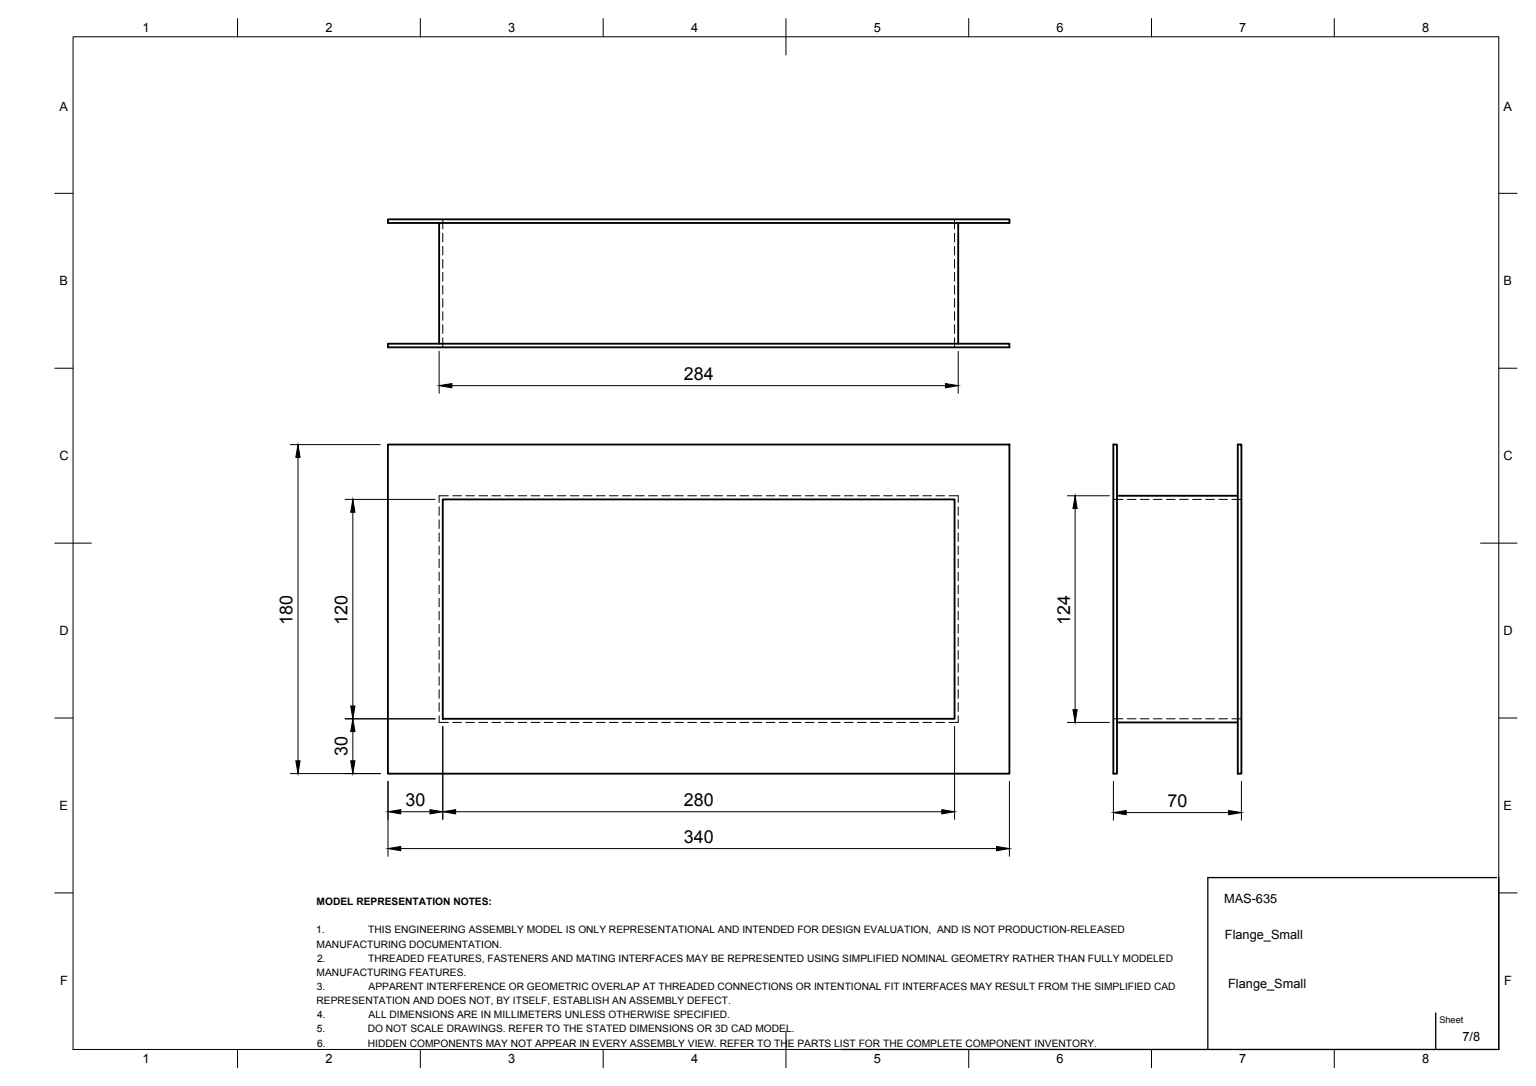
ISO-10303-21;
HEADER;
FILE_DESCRIPTION((''),'2;1');
FILE_NAME('Flange_Small.step','2026-10-09T12:34:24-07:00',(''),(''),'','','');
FILE_SCHEMA (('AUTOMOTIVE_DESIGN { 1 0 10303 214 3 1 1 }'));
ENDSEC;
DATA;
#10=MECHANICAL_DESIGN_GEOMETRIC_PRESENTATION_REPRESENTATION('',(#64),#3759);
#52=SHAPE_REPRESENTATION_RELATIONSHIP('SRR','None',#3793,#58) ;
#58=ADVANCED_BREP_SHAPE_REPRESENTATION('',(#70),#3758) ;
#64=STYLED_ITEM('',(#3827),#70) ;
#70=MANIFOLD_SOLID_BREP('Body1',#2268) ;
#137=FACE_BOUND('',#384,.T.) ;
#138=FACE_BOUND('',#386,.T.) ;
#139=FACE_BOUND('',#396,.T.) ;
#140=FACE_BOUND('',#398,.T.) ;
#241=FACE_OUTER_BOUND('',#379,.T.) ;
#242=FACE_OUTER_BOUND('',#380,.T.) ;
#243=FACE_OUTER_BOUND('',#381,.T.) ;
#244=FACE_OUTER_BOUND('',#382,.T.) ;
#245=FACE_OUTER_BOUND('',#383,.T.) ;
#246=FACE_OUTER_BOUND('',#385,.T.) ;
#247=FACE_OUTER_BOUND('',#387,.T.) ;
#248=FACE_OUTER_BOUND('',#388,.T.) ;
#249=FACE_OUTER_BOUND('',#389,.T.) ;
#250=FACE_OUTER_BOUND('',#390,.T.) ;
#251=FACE_OUTER_BOUND('',#391,.T.) ;
#252=FACE_OUTER_BOUND('',#392,.T.) ;
#253=FACE_OUTER_BOUND('',#393,.T.) ;
#254=FACE_OUTER_BOUND('',#394,.T.) ;
#255=FACE_OUTER_BOUND('',#395,.T.) ;
#256=FACE_OUTER_BOUND('',#397,.T.) ;
#257=FACE_OUTER_BOUND('',#399,.T.) ;
#258=FACE_OUTER_BOUND('',#400,.T.) ;
#259=FACE_OUTER_BOUND('',#401,.T.) ;
#260=FACE_OUTER_BOUND('',#402,.T.) ;
#379=EDGE_LOOP('',(#1943,#1944,#1945,#1946)) ;
#380=EDGE_LOOP('',(#1947,#1948,#1949,#1950)) ;
#381=EDGE_LOOP('',(#1951,#1952,#1953,#1954)) ;
#382=EDGE_LOOP('',(#1955,#1956,#1957,#1958)) ;
#383=EDGE_LOOP('',(#1959,#1960,#1961,#1962)) ;
#384=EDGE_LOOP('',(#1963,#1964,#1965,#1966)) ;
#385=EDGE_LOOP('',(#1967,#1968,#1969,#1970)) ;
#386=EDGE_LOOP('',(#1971,#1972,#1973,#1974)) ;
#387=EDGE_LOOP('',(#1975,#1976,#1977,#1978)) ;
#388=EDGE_LOOP('',(#1979,#1980,#1981,#1982)) ;
#389=EDGE_LOOP('',(#1983,#1984,#1985,#1986)) ;
#390=EDGE_LOOP('',(#1987,#1988,#1989,#1990)) ;
#391=EDGE_LOOP('',(#1991,#1992,#1993,#1994)) ;
#392=EDGE_LOOP('',(#1995,#1996,#1997,#1998)) ;
#393=EDGE_LOOP('',(#1999,#2000,#2001,#2002)) ;
#394=EDGE_LOOP('',(#2003,#2004,#2005,#2006)) ;
#395=EDGE_LOOP('',(#2007,#2008,#2009,#2010)) ;
#396=EDGE_LOOP('',(#2011,#2012,#2013,#2014)) ;
#397=EDGE_LOOP('',(#2015,#2016,#2017,#2018)) ;
#398=EDGE_LOOP('',(#2019,#2020,#2021,#2022)) ;
#399=EDGE_LOOP('',(#2023,#2024,#2025,#2026)) ;
#400=EDGE_LOOP('',(#2027,#2028,#2029,#2030)) ;
#401=EDGE_LOOP('',(#2031,#2032,#2033,#2034)) ;
#402=EDGE_LOOP('',(#2035,#2036,#2037,#2038)) ;
#623=LINE('',#3638,#891) ;
#624=LINE('',#3640,#892) ;
#625=LINE('',#3642,#893) ;
#626=LINE('',#3643,#894) ;
#627=LINE('',#3646,#895) ;
#628=LINE('',#3648,#896) ;
#629=LINE('',#3649,#897) ;
#630=LINE('',#3652,#898) ;
#631=LINE('',#3654,#899) ;
#632=LINE('',#3655,#900) ;
#633=LINE('',#3657,#901) ;
#634=LINE('',#3658,#902) ;
#635=LINE('',#3662,#903) ;
#636=LINE('',#3664,#904) ;
#637=LINE('',#3666,#905) ;
#638=LINE('',#3667,#906) ;
#639=LINE('',#3671,#907) ;
#640=LINE('',#3673,#908) ;
#641=LINE('',#3675,#909) ;
#642=LINE('',#3676,#910) ;
#643=LINE('',#3679,#911) ;
#644=LINE('',#3681,#912) ;
#645=LINE('',#3683,#913) ;
#646=LINE('',#3684,#914) ;
#647=LINE('',#3686,#915) ;
#648=LINE('',#3687,#916) ;
#649=LINE('',#3689,#917) ;
#650=LINE('',#3691,#918) ;
#651=LINE('',#3695,#919) ;
#652=LINE('',#3697,#920) ;
#653=LINE('',#3698,#921) ;
#654=LINE('',#3701,#922) ;
#655=LINE('',#3702,#923) ;
#656=LINE('',#3705,#924) ;
#657=LINE('',#3706,#925) ;
#658=LINE('',#3708,#926) ;
#659=LINE('',#3712,#927) ;
#660=LINE('',#3714,#928) ;
#661=LINE('',#3716,#929) ;
#662=LINE('',#3717,#930) ;
#663=LINE('',#3721,#931) ;
#664=LINE('',#3723,#932) ;
#665=LINE('',#3725,#933) ;
#666=LINE('',#3726,#934) ;
#667=LINE('',#3728,#935) ;
#668=LINE('',#3729,#936) ;
#669=LINE('',#3731,#937) ;
#670=LINE('',#3733,#938) ;
#891=VECTOR('',#3004,100.) ;
#892=VECTOR('',#3005,100.) ;
#893=VECTOR('',#3006,100.) ;
#894=VECTOR('',#3007,100.) ;
#895=VECTOR('',#3010,100.) ;
#896=VECTOR('',#3011,100.) ;
#897=VECTOR('',#3012,100.) ;
#898=VECTOR('',#3015,100.) ;
#899=VECTOR('',#3016,100.) ;
#900=VECTOR('',#3017,100.) ;
#901=VECTOR('',#3020,100.) ;
#902=VECTOR('',#3021,100.) ;
#903=VECTOR('',#3024,100.) ;
#904=VECTOR('',#3025,100.) ;
#905=VECTOR('',#3026,100.) ;
#906=VECTOR('',#3027,100.) ;
#907=VECTOR('',#3030,100.) ;
#908=VECTOR('',#3031,100.) ;
#909=VECTOR('',#3032,100.) ;
#910=VECTOR('',#3033,100.) ;
#911=VECTOR('',#3034,100.) ;
#912=VECTOR('',#3035,100.) ;
#913=VECTOR('',#3036,100.) ;
#914=VECTOR('',#3037,100.) ;
#915=VECTOR('',#3040,100.) ;
#916=VECTOR('',#3041,100.) ;
#917=VECTOR('',#3044,100.) ;
#918=VECTOR('',#3047,100.) ;
#919=VECTOR('',#3052,100.) ;
#920=VECTOR('',#3053,100.) ;
#921=VECTOR('',#3054,100.) ;
#922=VECTOR('',#3057,100.) ;
#923=VECTOR('',#3058,100.) ;
#924=VECTOR('',#3061,100.) ;
#925=VECTOR('',#3062,100.) ;
#926=VECTOR('',#3065,100.) ;
#927=VECTOR('',#3068,100.) ;
#928=VECTOR('',#3069,100.) ;
#929=VECTOR('',#3070,100.) ;
#930=VECTOR('',#3071,100.) ;
#931=VECTOR('',#3074,100.) ;
#932=VECTOR('',#3075,100.) ;
#933=VECTOR('',#3076,100.) ;
#934=VECTOR('',#3077,100.) ;
#935=VECTOR('',#3080,100.) ;
#936=VECTOR('',#3081,100.) ;
#937=VECTOR('',#3084,100.) ;
#938=VECTOR('',#3087,100.) ;
#1107=VERTEX_POINT('',#3636) ;
#1108=VERTEX_POINT('',#3637) ;
#1109=VERTEX_POINT('',#3639) ;
#1110=VERTEX_POINT('',#3641) ;
#1111=VERTEX_POINT('',#3645) ;
#1112=VERTEX_POINT('',#3647) ;
#1113=VERTEX_POINT('',#3651) ;
#1114=VERTEX_POINT('',#3653) ;
#1115=VERTEX_POINT('',#3660) ;
#1116=VERTEX_POINT('',#3661) ;
#1117=VERTEX_POINT('',#3663) ;
#1118=VERTEX_POINT('',#3665) ;
#1119=VERTEX_POINT('',#3669) ;
#1120=VERTEX_POINT('',#3670) ;
#1121=VERTEX_POINT('',#3672) ;
#1122=VERTEX_POINT('',#3674) ;
#1123=VERTEX_POINT('',#3677) ;
#1124=VERTEX_POINT('',#3678) ;
#1125=VERTEX_POINT('',#3680) ;
#1126=VERTEX_POINT('',#3682) ;
#1127=VERTEX_POINT('',#3694) ;
#1128=VERTEX_POINT('',#3696) ;
#1129=VERTEX_POINT('',#3700) ;
#1130=VERTEX_POINT('',#3704) ;
#1131=VERTEX_POINT('',#3710) ;
#1132=VERTEX_POINT('',#3711) ;
#1133=VERTEX_POINT('',#3713) ;
#1134=VERTEX_POINT('',#3715) ;
#1135=VERTEX_POINT('',#3719) ;
#1136=VERTEX_POINT('',#3720) ;
#1137=VERTEX_POINT('',#3722) ;
#1138=VERTEX_POINT('',#3724) ;
#1391=EDGE_CURVE('',#1107,#1108,#623,.T.) ;
#1392=EDGE_CURVE('',#1107,#1109,#624,.T.) ;
#1393=EDGE_CURVE('',#1110,#1109,#625,.T.) ;
#1394=EDGE_CURVE('',#1108,#1110,#626,.T.) ;
#1395=EDGE_CURVE('',#1108,#1111,#627,.T.) ;
#1396=EDGE_CURVE('',#1112,#1110,#628,.T.) ;
#1397=EDGE_CURVE('',#1111,#1112,#629,.T.) ;
#1398=EDGE_CURVE('',#1111,#1113,#630,.T.) ;
#1399=EDGE_CURVE('',#1114,#1112,#631,.T.) ;
#1400=EDGE_CURVE('',#1113,#1114,#632,.T.) ;
#1401=EDGE_CURVE('',#1113,#1107,#633,.T.) ;
#1402=EDGE_CURVE('',#1109,#1114,#634,.T.) ;
#1403=EDGE_CURVE('',#1115,#1116,#635,.T.) ;
#1404=EDGE_CURVE('',#1116,#1117,#636,.T.) ;
#1405=EDGE_CURVE('',#1117,#1118,#637,.T.) ;
#1406=EDGE_CURVE('',#1118,#1115,#638,.T.) ;
#1407=EDGE_CURVE('',#1119,#1120,#639,.T.) ;
#1408=EDGE_CURVE('',#1121,#1119,#640,.T.) ;
#1409=EDGE_CURVE('',#1122,#1121,#641,.T.) ;
#1410=EDGE_CURVE('',#1120,#1122,#642,.T.) ;
#1411=EDGE_CURVE('',#1123,#1124,#643,.T.) ;
#1412=EDGE_CURVE('',#1124,#1125,#644,.T.) ;
#1413=EDGE_CURVE('',#1125,#1126,#645,.T.) ;
#1414=EDGE_CURVE('',#1126,#1123,#646,.T.) ;
#1415=EDGE_CURVE('',#1116,#1120,#647,.T.) ;
#1416=EDGE_CURVE('',#1115,#1119,#648,.T.) ;
#1417=EDGE_CURVE('',#1117,#1122,#649,.T.) ;
#1418=EDGE_CURVE('',#1118,#1121,#650,.T.) ;
#1419=EDGE_CURVE('',#1127,#1124,#651,.T.) ;
#1420=EDGE_CURVE('',#1128,#1123,#652,.T.) ;
#1421=EDGE_CURVE('',#1128,#1127,#653,.T.) ;
#1422=EDGE_CURVE('',#1129,#1125,#654,.T.) ;
#1423=EDGE_CURVE('',#1127,#1129,#655,.T.) ;
#1424=EDGE_CURVE('',#1130,#1126,#656,.T.) ;
#1425=EDGE_CURVE('',#1129,#1130,#657,.T.) ;
#1426=EDGE_CURVE('',#1130,#1128,#658,.T.) ;
#1427=EDGE_CURVE('',#1131,#1132,#659,.T.) ;
#1428=EDGE_CURVE('',#1132,#1133,#660,.T.) ;
#1429=EDGE_CURVE('',#1133,#1134,#661,.T.) ;
#1430=EDGE_CURVE('',#1134,#1131,#662,.T.) ;
#1431=EDGE_CURVE('',#1135,#1136,#663,.T.) ;
#1432=EDGE_CURVE('',#1137,#1135,#664,.T.) ;
#1433=EDGE_CURVE('',#1138,#1137,#665,.T.) ;
#1434=EDGE_CURVE('',#1136,#1138,#666,.T.) ;
#1435=EDGE_CURVE('',#1135,#1131,#667,.T.) ;
#1436=EDGE_CURVE('',#1136,#1132,#668,.T.) ;
#1437=EDGE_CURVE('',#1137,#1134,#669,.T.) ;
#1438=EDGE_CURVE('',#1138,#1133,#670,.T.) ;
#1943=ORIENTED_EDGE('',*,*,#1391,.F.) ;
#1944=ORIENTED_EDGE('',*,*,#1392,.T.) ;
#1945=ORIENTED_EDGE('',*,*,#1393,.F.) ;
#1946=ORIENTED_EDGE('',*,*,#1394,.F.) ;
#1947=ORIENTED_EDGE('',*,*,#1395,.F.) ;
#1948=ORIENTED_EDGE('',*,*,#1394,.T.) ;
#1949=ORIENTED_EDGE('',*,*,#1396,.F.) ;
#1950=ORIENTED_EDGE('',*,*,#1397,.F.) ;
#1951=ORIENTED_EDGE('',*,*,#1398,.F.) ;
#1952=ORIENTED_EDGE('',*,*,#1397,.T.) ;
#1953=ORIENTED_EDGE('',*,*,#1399,.F.) ;
#1954=ORIENTED_EDGE('',*,*,#1400,.F.) ;
#1955=ORIENTED_EDGE('',*,*,#1401,.F.) ;
#1956=ORIENTED_EDGE('',*,*,#1400,.T.) ;
#1957=ORIENTED_EDGE('',*,*,#1402,.F.) ;
#1958=ORIENTED_EDGE('',*,*,#1392,.F.) ;
#1959=ORIENTED_EDGE('',*,*,#1403,.T.) ;
#1960=ORIENTED_EDGE('',*,*,#1404,.T.) ;
#1961=ORIENTED_EDGE('',*,*,#1405,.T.) ;
#1962=ORIENTED_EDGE('',*,*,#1406,.T.) ;
#1963=ORIENTED_EDGE('',*,*,#1396,.T.) ;
#1964=ORIENTED_EDGE('',*,*,#1393,.T.) ;
#1965=ORIENTED_EDGE('',*,*,#1402,.T.) ;
#1966=ORIENTED_EDGE('',*,*,#1399,.T.) ;
#1967=ORIENTED_EDGE('',*,*,#1407,.F.) ;
#1968=ORIENTED_EDGE('',*,*,#1408,.F.) ;
#1969=ORIENTED_EDGE('',*,*,#1409,.F.) ;
#1970=ORIENTED_EDGE('',*,*,#1410,.F.) ;
#1971=ORIENTED_EDGE('',*,*,#1411,.T.) ;
#1972=ORIENTED_EDGE('',*,*,#1412,.T.) ;
#1973=ORIENTED_EDGE('',*,*,#1413,.T.) ;
#1974=ORIENTED_EDGE('',*,*,#1414,.T.) ;
#1975=ORIENTED_EDGE('',*,*,#1407,.T.) ;
#1976=ORIENTED_EDGE('',*,*,#1415,.F.) ;
#1977=ORIENTED_EDGE('',*,*,#1403,.F.) ;
#1978=ORIENTED_EDGE('',*,*,#1416,.T.) ;
#1979=ORIENTED_EDGE('',*,*,#1410,.T.) ;
#1980=ORIENTED_EDGE('',*,*,#1417,.F.) ;
#1981=ORIENTED_EDGE('',*,*,#1404,.F.) ;
#1982=ORIENTED_EDGE('',*,*,#1415,.T.) ;
#1983=ORIENTED_EDGE('',*,*,#1409,.T.) ;
#1984=ORIENTED_EDGE('',*,*,#1418,.F.) ;
#1985=ORIENTED_EDGE('',*,*,#1405,.F.) ;
#1986=ORIENTED_EDGE('',*,*,#1417,.T.) ;
#1987=ORIENTED_EDGE('',*,*,#1408,.T.) ;
#1988=ORIENTED_EDGE('',*,*,#1416,.F.) ;
#1989=ORIENTED_EDGE('',*,*,#1406,.F.) ;
#1990=ORIENTED_EDGE('',*,*,#1418,.T.) ;
#1991=ORIENTED_EDGE('',*,*,#1419,.T.) ;
#1992=ORIENTED_EDGE('',*,*,#1411,.F.) ;
#1993=ORIENTED_EDGE('',*,*,#1420,.F.) ;
#1994=ORIENTED_EDGE('',*,*,#1421,.T.) ;
#1995=ORIENTED_EDGE('',*,*,#1422,.T.) ;
#1996=ORIENTED_EDGE('',*,*,#1412,.F.) ;
#1997=ORIENTED_EDGE('',*,*,#1419,.F.) ;
#1998=ORIENTED_EDGE('',*,*,#1423,.T.) ;
#1999=ORIENTED_EDGE('',*,*,#1424,.T.) ;
#2000=ORIENTED_EDGE('',*,*,#1413,.F.) ;
#2001=ORIENTED_EDGE('',*,*,#1422,.F.) ;
#2002=ORIENTED_EDGE('',*,*,#1425,.T.) ;
#2003=ORIENTED_EDGE('',*,*,#1420,.T.) ;
#2004=ORIENTED_EDGE('',*,*,#1414,.F.) ;
#2005=ORIENTED_EDGE('',*,*,#1424,.F.) ;
#2006=ORIENTED_EDGE('',*,*,#1426,.T.) ;
#2007=ORIENTED_EDGE('',*,*,#1427,.T.) ;
#2008=ORIENTED_EDGE('',*,*,#1428,.T.) ;
#2009=ORIENTED_EDGE('',*,*,#1429,.T.) ;
#2010=ORIENTED_EDGE('',*,*,#1430,.T.) ;
#2011=ORIENTED_EDGE('',*,*,#1423,.F.) ;
#2012=ORIENTED_EDGE('',*,*,#1421,.F.) ;
#2013=ORIENTED_EDGE('',*,*,#1426,.F.) ;
#2014=ORIENTED_EDGE('',*,*,#1425,.F.) ;
#2015=ORIENTED_EDGE('',*,*,#1431,.F.) ;
#2016=ORIENTED_EDGE('',*,*,#1432,.F.) ;
#2017=ORIENTED_EDGE('',*,*,#1433,.F.) ;
#2018=ORIENTED_EDGE('',*,*,#1434,.F.) ;
#2019=ORIENTED_EDGE('',*,*,#1401,.T.) ;
#2020=ORIENTED_EDGE('',*,*,#1391,.T.) ;
#2021=ORIENTED_EDGE('',*,*,#1395,.T.) ;
#2022=ORIENTED_EDGE('',*,*,#1398,.T.) ;
#2023=ORIENTED_EDGE('',*,*,#1427,.F.) ;
#2024=ORIENTED_EDGE('',*,*,#1435,.F.) ;
#2025=ORIENTED_EDGE('',*,*,#1431,.T.) ;
#2026=ORIENTED_EDGE('',*,*,#1436,.T.) ;
#2027=ORIENTED_EDGE('',*,*,#1430,.F.) ;
#2028=ORIENTED_EDGE('',*,*,#1437,.F.) ;
#2029=ORIENTED_EDGE('',*,*,#1432,.T.) ;
#2030=ORIENTED_EDGE('',*,*,#1435,.T.) ;
#2031=ORIENTED_EDGE('',*,*,#1429,.F.) ;
#2032=ORIENTED_EDGE('',*,*,#1438,.F.) ;
#2033=ORIENTED_EDGE('',*,*,#1433,.T.) ;
#2034=ORIENTED_EDGE('',*,*,#1437,.T.) ;
#2035=ORIENTED_EDGE('',*,*,#1428,.F.) ;
#2036=ORIENTED_EDGE('',*,*,#1436,.F.) ;
#2037=ORIENTED_EDGE('',*,*,#1434,.T.) ;
#2038=ORIENTED_EDGE('',*,*,#1438,.T.) ;
#2123=PLANE('',#2475) ;
#2124=PLANE('',#2476) ;
#2125=PLANE('',#2477) ;
#2126=PLANE('',#2478) ;
#2127=PLANE('',#2479) ;
#2128=PLANE('',#2480) ;
#2129=PLANE('',#2481) ;
#2130=PLANE('',#2482) ;
#2131=PLANE('',#2483) ;
#2132=PLANE('',#2484) ;
#2133=PLANE('',#2485) ;
#2134=PLANE('',#2486) ;
#2135=PLANE('',#2487) ;
#2136=PLANE('',#2488) ;
#2137=PLANE('',#2489) ;
#2138=PLANE('',#2490) ;
#2139=PLANE('',#2491) ;
#2140=PLANE('',#2492) ;
#2141=PLANE('',#2493) ;
#2142=PLANE('',#2494) ;
#2243=ADVANCED_FACE('',(#241),#2123,.F.) ;
#2244=ADVANCED_FACE('',(#242),#2124,.F.) ;
#2245=ADVANCED_FACE('',(#243),#2125,.F.) ;
#2246=ADVANCED_FACE('',(#244),#2126,.F.) ;
#2247=ADVANCED_FACE('',(#245,#137),#2127,.T.) ;
#2248=ADVANCED_FACE('',(#246,#138),#2128,.F.) ;
#2249=ADVANCED_FACE('',(#247),#2129,.F.) ;
#2250=ADVANCED_FACE('',(#248),#2130,.F.) ;
#2251=ADVANCED_FACE('',(#249),#2131,.F.) ;
#2252=ADVANCED_FACE('',(#250),#2132,.F.) ;
#2253=ADVANCED_FACE('',(#251),#2133,.T.) ;
#2254=ADVANCED_FACE('',(#252),#2134,.T.) ;
#2255=ADVANCED_FACE('',(#253),#2135,.T.) ;
#2256=ADVANCED_FACE('',(#254),#2136,.T.) ;
#2257=ADVANCED_FACE('',(#255,#139),#2137,.T.) ;
#2258=ADVANCED_FACE('',(#256,#140),#2138,.F.) ;
#2259=ADVANCED_FACE('',(#257),#2139,.T.) ;
#2260=ADVANCED_FACE('',(#258),#2140,.T.) ;
#2261=ADVANCED_FACE('',(#259),#2141,.T.) ;
#2262=ADVANCED_FACE('',(#260),#2142,.T.) ;
#2268=CLOSED_SHELL('',(#2243,#2244,#2245,#2246,#2247,#2248,#2249,#2250,
#2251,#2252,#2253,#2254,#2255,#2256,#2257,#2258,#2259,#2260,#2261,#2262)) ;
#2474=AXIS2_PLACEMENT_3D('',#3634,#3000,#3001) ;
#2475=AXIS2_PLACEMENT_3D('',#3635,#3002,#3003) ;
#2476=AXIS2_PLACEMENT_3D('',#3644,#3008,#3009) ;
#2477=AXIS2_PLACEMENT_3D('',#3650,#3013,#3014) ;
#2478=AXIS2_PLACEMENT_3D('',#3656,#3018,#3019) ;
#2479=AXIS2_PLACEMENT_3D('',#3659,#3022,#3023) ;
#2480=AXIS2_PLACEMENT_3D('',#3668,#3028,#3029) ;
#2481=AXIS2_PLACEMENT_3D('',#3685,#3038,#3039) ;
#2482=AXIS2_PLACEMENT_3D('',#3688,#3042,#3043) ;
#2483=AXIS2_PLACEMENT_3D('',#3690,#3045,#3046) ;
#2484=AXIS2_PLACEMENT_3D('',#3692,#3048,#3049) ;
#2485=AXIS2_PLACEMENT_3D('',#3693,#3050,#3051) ;
#2486=AXIS2_PLACEMENT_3D('',#3699,#3055,#3056) ;
#2487=AXIS2_PLACEMENT_3D('',#3703,#3059,#3060) ;
#2488=AXIS2_PLACEMENT_3D('',#3707,#3063,#3064) ;
#2489=AXIS2_PLACEMENT_3D('',#3709,#3066,#3067) ;
#2490=AXIS2_PLACEMENT_3D('',#3718,#3072,#3073) ;
#2491=AXIS2_PLACEMENT_3D('',#3727,#3078,#3079) ;
#2492=AXIS2_PLACEMENT_3D('',#3730,#3082,#3083) ;
#2493=AXIS2_PLACEMENT_3D('',#3732,#3085,#3086) ;
#2494=AXIS2_PLACEMENT_3D('',#3734,#3088,#3089) ;
#3000=DIRECTION('axis',(0.,0.,1.)) ;
#3001=DIRECTION('refdir',(1.,0.,0.)) ;
#3002=DIRECTION('center_axis',(-1.,4.62592926927149E-16,0.)) ;
#3003=DIRECTION('ref_axis',(-4.62592926927149E-16,-1.,0.)) ;
#3004=DIRECTION('',(4.62592926927149E-16,1.,0.)) ;
#3005=DIRECTION('',(0.,0.,-1.)) ;
#3006=DIRECTION('',(-4.62592926927149E-16,-1.,0.)) ;
#3007=DIRECTION('',(0.,0.,-1.)) ;
#3008=DIRECTION('center_axis',(0.,-1.,0.)) ;
#3009=DIRECTION('ref_axis',(0.,0.,-1.)) ;
#3010=DIRECTION('',(-1.,0.,0.)) ;
#3011=DIRECTION('',(1.,0.,0.)) ;
#3012=DIRECTION('',(0.,0.,-1.)) ;
#3013=DIRECTION('center_axis',(1.,-4.62592926927149E-16,0.)) ;
#3014=DIRECTION('ref_axis',(4.62592926927149E-16,1.,0.)) ;
#3015=DIRECTION('',(-4.62592926927149E-16,-1.,0.)) ;
#3016=DIRECTION('',(4.62592926927149E-16,1.,0.)) ;
#3017=DIRECTION('',(0.,0.,-1.)) ;
#3018=DIRECTION('center_axis',(0.,1.,0.)) ;
#3019=DIRECTION('ref_axis',(0.,0.,1.)) ;
#3020=DIRECTION('',(1.,0.,0.)) ;
#3021=DIRECTION('',(-1.,0.,0.)) ;
#3022=DIRECTION('center_axis',(0.,0.,1.)) ;
#3023=DIRECTION('ref_axis',(1.,0.,0.)) ;
#3024=DIRECTION('',(4.62592926927149E-16,1.,0.)) ;
#3025=DIRECTION('',(-1.,0.,0.)) ;
#3026=DIRECTION('',(-4.62592926927149E-16,-1.,0.)) ;
#3027=DIRECTION('',(1.,0.,0.)) ;
#3028=DIRECTION('center_axis',(0.,0.,1.)) ;
#3029=DIRECTION('ref_axis',(1.,0.,0.)) ;
#3030=DIRECTION('',(4.62592926927149E-16,1.,0.)) ;
#3031=DIRECTION('',(1.,0.,0.)) ;
#3032=DIRECTION('',(-4.62592926927149E-16,-1.,0.)) ;
#3033=DIRECTION('',(-1.,0.,0.)) ;
#3034=DIRECTION('',(4.62592926927149E-16,1.,0.)) ;
#3035=DIRECTION('',(-1.,0.,0.)) ;
#3036=DIRECTION('',(-4.62592926927149E-16,-1.,0.)) ;
#3037=DIRECTION('',(1.,0.,0.)) ;
#3038=DIRECTION('center_axis',(-1.,4.62592926927149E-16,0.)) ;
#3039=DIRECTION('ref_axis',(-4.62592926927149E-16,-1.,0.)) ;
#3040=DIRECTION('',(0.,0.,-1.)) ;
#3041=DIRECTION('',(0.,0.,-1.)) ;
#3042=DIRECTION('center_axis',(0.,-1.,0.)) ;
#3043=DIRECTION('ref_axis',(0.,0.,-1.)) ;
#3044=DIRECTION('',(0.,0.,-1.)) ;
#3045=DIRECTION('center_axis',(1.,-4.62592926927149E-16,0.)) ;
#3046=DIRECTION('ref_axis',(4.62592926927149E-16,1.,0.)) ;
#3047=DIRECTION('',(0.,0.,-1.)) ;
#3048=DIRECTION('center_axis',(0.,1.,0.)) ;
#3049=DIRECTION('ref_axis',(0.,0.,1.)) ;
#3050=DIRECTION('center_axis',(-1.,4.62592926927149E-16,0.)) ;
#3051=DIRECTION('ref_axis',(-4.62592926927149E-16,-1.,0.)) ;
#3052=DIRECTION('',(0.,0.,-1.)) ;
#3053=DIRECTION('',(0.,0.,-1.)) ;
#3054=DIRECTION('',(4.62592926927149E-16,1.,0.)) ;
#3055=DIRECTION('center_axis',(0.,-1.,0.)) ;
#3056=DIRECTION('ref_axis',(0.,0.,-1.)) ;
#3057=DIRECTION('',(0.,0.,-1.)) ;
#3058=DIRECTION('',(-1.,0.,0.)) ;
#3059=DIRECTION('center_axis',(1.,-4.62592926927149E-16,0.)) ;
#3060=DIRECTION('ref_axis',(4.62592926927149E-16,1.,0.)) ;
#3061=DIRECTION('',(0.,0.,-1.)) ;
#3062=DIRECTION('',(-4.62592926927149E-16,-1.,0.)) ;
#3063=DIRECTION('center_axis',(0.,1.,0.)) ;
#3064=DIRECTION('ref_axis',(0.,0.,1.)) ;
#3065=DIRECTION('',(1.,0.,0.)) ;
#3066=DIRECTION('center_axis',(0.,0.,1.)) ;
#3067=DIRECTION('ref_axis',(1.,0.,0.)) ;
#3068=DIRECTION('',(-4.62592926927149E-16,-1.,0.)) ;
#3069=DIRECTION('',(1.,0.,0.)) ;
#3070=DIRECTION('',(4.62592926927149E-16,1.,0.)) ;
#3071=DIRECTION('',(-1.,0.,0.)) ;
#3072=DIRECTION('center_axis',(0.,0.,1.)) ;
#3073=DIRECTION('ref_axis',(1.,0.,0.)) ;
#3074=DIRECTION('',(-4.62592926927149E-16,-1.,0.)) ;
#3075=DIRECTION('',(-1.,0.,0.)) ;
#3076=DIRECTION('',(4.62592926927149E-16,1.,0.)) ;
#3077=DIRECTION('',(1.,0.,0.)) ;
#3078=DIRECTION('center_axis',(-1.,4.62592926927149E-16,0.)) ;
#3079=DIRECTION('ref_axis',(-4.62592926927149E-16,-1.,0.)) ;
#3080=DIRECTION('',(0.,0.,1.)) ;
#3081=DIRECTION('',(0.,0.,1.)) ;
#3082=DIRECTION('center_axis',(0.,1.,0.)) ;
#3083=DIRECTION('ref_axis',(0.,0.,1.)) ;
#3084=DIRECTION('',(0.,0.,1.)) ;
#3085=DIRECTION('center_axis',(1.,-4.62592926927149E-16,0.)) ;
#3086=DIRECTION('ref_axis',(4.62592926927149E-16,1.,0.)) ;
#3087=DIRECTION('',(0.,0.,1.)) ;
#3088=DIRECTION('center_axis',(0.,-1.,0.)) ;
#3089=DIRECTION('ref_axis',(0.,0.,-1.)) ;
#3634=CARTESIAN_POINT('',(0.,0.,0.)) ;
#3635=CARTESIAN_POINT('Origin',(14.2,6.,7.)) ;
#3636=CARTESIAN_POINT('',(14.2,-6.2,6.8)) ;
#3637=CARTESIAN_POINT('',(14.2,6.2,6.8)) ;
#3638=CARTESIAN_POINT('',(14.2,6.,6.8)) ;
#3639=CARTESIAN_POINT('',(14.2,-6.2,0.2)) ;
#3640=CARTESIAN_POINT('',(14.2,-6.2,7.)) ;
#3641=CARTESIAN_POINT('',(14.2,6.2,0.2)) ;
#3642=CARTESIAN_POINT('',(14.2,-6.56881956236551E-15,0.2)) ;
#3643=CARTESIAN_POINT('',(14.2,6.2,7.)) ;
#3644=CARTESIAN_POINT('Origin',(-14.,6.2,7.)) ;
#3645=CARTESIAN_POINT('',(-14.2,6.2,6.8)) ;
#3646=CARTESIAN_POINT('',(-14.,6.2,6.8)) ;
#3647=CARTESIAN_POINT('',(-14.2,6.2,0.2)) ;
#3648=CARTESIAN_POINT('',(0.,6.2,0.2)) ;
#3649=CARTESIAN_POINT('',(-14.2,6.2,7.)) ;
#3650=CARTESIAN_POINT('Origin',(-14.2,6.,7.)) ;
#3651=CARTESIAN_POINT('',(-14.2,-6.2,6.8)) ;
#3652=CARTESIAN_POINT('',(-14.2,6.,6.8)) ;
#3653=CARTESIAN_POINT('',(-14.2,-6.2,0.2)) ;
#3654=CARTESIAN_POINT('',(-14.2,6.56881956236551E-15,0.2)) ;
#3655=CARTESIAN_POINT('',(-14.2,-6.2,7.)) ;
#3656=CARTESIAN_POINT('Origin',(-14.,-6.2,7.)) ;
#3657=CARTESIAN_POINT('',(-14.,-6.2,6.8)) ;
#3658=CARTESIAN_POINT('',(0.,-6.2,0.2)) ;
#3659=CARTESIAN_POINT('Origin',(0.,0.,0.2)) ;
#3660=CARTESIAN_POINT('',(17.,-9.,0.2)) ;
#3661=CARTESIAN_POINT('',(17.,9.,0.2)) ;
#3662=CARTESIAN_POINT('',(17.,6.,0.2)) ;
#3663=CARTESIAN_POINT('',(-17.,9.,0.2)) ;
#3664=CARTESIAN_POINT('',(-14.,9.,0.2)) ;
#3665=CARTESIAN_POINT('',(-17.,-9.,0.2)) ;
#3666=CARTESIAN_POINT('',(-17.,6.,0.2)) ;
#3667=CARTESIAN_POINT('',(-14.,-9.,0.2)) ;
#3668=CARTESIAN_POINT('Origin',(0.,0.,0.)) ;
#3669=CARTESIAN_POINT('',(17.,-9.,0.)) ;
#3670=CARTESIAN_POINT('',(17.,9.,0.)) ;
#3671=CARTESIAN_POINT('',(17.,6.,0.)) ;
#3672=CARTESIAN_POINT('',(-17.,-9.,0.)) ;
#3673=CARTESIAN_POINT('',(-14.,-9.,0.)) ;
#3674=CARTESIAN_POINT('',(-17.,9.,0.)) ;
#3675=CARTESIAN_POINT('',(-17.,6.,0.)) ;
#3676=CARTESIAN_POINT('',(-14.,9.,0.)) ;
#3677=CARTESIAN_POINT('',(14.,-6.,0.)) ;
#3678=CARTESIAN_POINT('',(14.,6.,0.)) ;
#3679=CARTESIAN_POINT('',(14.,6.,0.)) ;
#3680=CARTESIAN_POINT('',(-14.,6.,0.)) ;
#3681=CARTESIAN_POINT('',(-14.,6.,0.)) ;
#3682=CARTESIAN_POINT('',(-14.,-6.,0.)) ;
#3683=CARTESIAN_POINT('',(-14.,6.,0.)) ;
#3684=CARTESIAN_POINT('',(-14.,-6.,0.)) ;
#3685=CARTESIAN_POINT('Origin',(17.,6.,0.2)) ;
#3686=CARTESIAN_POINT('',(17.,9.,0.2)) ;
#3687=CARTESIAN_POINT('',(17.,-9.,0.2)) ;
#3688=CARTESIAN_POINT('Origin',(-14.,9.,0.2)) ;
#3689=CARTESIAN_POINT('',(-17.,9.,0.2)) ;
#3690=CARTESIAN_POINT('Origin',(-17.,6.,0.2)) ;
#3691=CARTESIAN_POINT('',(-17.,-9.,0.2)) ;
#3692=CARTESIAN_POINT('Origin',(-14.,-9.,0.2)) ;
#3693=CARTESIAN_POINT('Origin',(14.,6.,0.2)) ;
#3694=CARTESIAN_POINT('',(14.,6.,7.)) ;
#3695=CARTESIAN_POINT('',(14.,6.,0.2)) ;
#3696=CARTESIAN_POINT('',(14.,-6.,7.)) ;
#3697=CARTESIAN_POINT('',(14.,-6.,0.2)) ;
#3698=CARTESIAN_POINT('',(14.,6.,7.)) ;
#3699=CARTESIAN_POINT('Origin',(-14.,6.,0.2)) ;
#3700=CARTESIAN_POINT('',(-14.,6.,7.)) ;
#3701=CARTESIAN_POINT('',(-14.,6.,0.2)) ;
#3702=CARTESIAN_POINT('',(-14.,6.,7.)) ;
#3703=CARTESIAN_POINT('Origin',(-14.,6.,0.2)) ;
#3704=CARTESIAN_POINT('',(-14.,-6.,7.)) ;
#3705=CARTESIAN_POINT('',(-14.,-6.,0.2)) ;
#3706=CARTESIAN_POINT('',(-14.,6.,7.)) ;
#3707=CARTESIAN_POINT('Origin',(-14.,-6.,0.2)) ;
#3708=CARTESIAN_POINT('',(-14.,-6.,7.)) ;
#3709=CARTESIAN_POINT('Origin',(0.,0.,7.)) ;
#3710=CARTESIAN_POINT('',(-17.,9.,7.)) ;
#3711=CARTESIAN_POINT('',(-17.,-9.,7.)) ;
#3712=CARTESIAN_POINT('',(-17.,6.,7.)) ;
#3713=CARTESIAN_POINT('',(17.,-9.,7.)) ;
#3714=CARTESIAN_POINT('',(-14.,-9.,7.)) ;
#3715=CARTESIAN_POINT('',(17.,9.,7.)) ;
#3716=CARTESIAN_POINT('',(17.,-6.,7.)) ;
#3717=CARTESIAN_POINT('',(14.,9.,7.)) ;
#3718=CARTESIAN_POINT('Origin',(0.,0.,6.8)) ;
#3719=CARTESIAN_POINT('',(-17.,9.,6.8)) ;
#3720=CARTESIAN_POINT('',(-17.,-9.,6.8)) ;
#3721=CARTESIAN_POINT('',(-17.,6.,6.8)) ;
#3722=CARTESIAN_POINT('',(17.,9.,6.8)) ;
#3723=CARTESIAN_POINT('',(14.,9.,6.8)) ;
#3724=CARTESIAN_POINT('',(17.,-9.,6.8)) ;
#3725=CARTESIAN_POINT('',(17.,-6.,6.8)) ;
#3726=CARTESIAN_POINT('',(-14.,-9.,6.8)) ;
#3727=CARTESIAN_POINT('Origin',(-17.,6.,6.8)) ;
#3728=CARTESIAN_POINT('',(-17.,9.,6.8)) ;
#3729=CARTESIAN_POINT('',(-17.,-9.,6.8)) ;
#3730=CARTESIAN_POINT('Origin',(14.,9.,6.8)) ;
#3731=CARTESIAN_POINT('',(17.,9.,6.8)) ;
#3732=CARTESIAN_POINT('Origin',(17.,-6.,6.8)) ;
#3733=CARTESIAN_POINT('',(17.,-9.,6.8)) ;
#3734=CARTESIAN_POINT('Origin',(-14.,-9.,6.8)) ;
#3750=UNCERTAINTY_MEASURE_WITH_UNIT(LENGTH_MEASURE(0.001),#3760,
'DISTANCE_ACCURACY_VALUE',
'Maximum model space distance between geometric entities at asserted c
onnectivities') ;
#3751=UNCERTAINTY_MEASURE_WITH_UNIT(LENGTH_MEASURE(0.001),#3760,
'DISTANCE_ACCURACY_VALUE',
'Maximum model space distance between geometric entities at asserted c
onnectivities') ;
#3758=(
GEOMETRIC_REPRESENTATION_CONTEXT(3)
GLOBAL_UNCERTAINTY_ASSIGNED_CONTEXT((#3750))
GLOBAL_UNIT_ASSIGNED_CONTEXT((#3760,#3762,#3763))
REPRESENTATION_CONTEXT('','3D')
) ;
#3759=(
GEOMETRIC_REPRESENTATION_CONTEXT(3)
GLOBAL_UNCERTAINTY_ASSIGNED_CONTEXT((#3751))
GLOBAL_UNIT_ASSIGNED_CONTEXT((#3760,#3762,#3763))
REPRESENTATION_CONTEXT('','3D')
) ;
#3760=(
LENGTH_UNIT()
NAMED_UNIT(*)
SI_UNIT(.CENTI.,.METRE.)
) ;
#3762=(
NAMED_UNIT(*)
PLANE_ANGLE_UNIT()
SI_UNIT($,.RADIAN.)
) ;
#3763=(
NAMED_UNIT(*)
SI_UNIT($,.STERADIAN.)
SOLID_ANGLE_UNIT()
) ;
#3770=SHAPE_DEFINITION_REPRESENTATION(#3777,#3793) ;
#3777=PRODUCT_DEFINITION_SHAPE('',$,#3801) ;
#3793=SHAPE_REPRESENTATION('',(#2474),#3758) ;
#3794=PRODUCT_DEFINITION_CONTEXT('part definition',#3817,'design') ;
#3801=PRODUCT_DEFINITION('Flange_Small','Flange_Small',#3808,
#3794) ;
#3808=PRODUCT_DEFINITION_FORMATION('',$,#3825) ;
#3817=APPLICATION_CONTEXT(
'Core Data for Automotive Mechanical Design Process') ;
#3818=PRODUCT_CONTEXT('part definition',#3817,'mechanical') ;
#3825=PRODUCT('Flange_Small','Flange_Small',$,(#3818)) ;
#3827=PRESENTATION_STYLE_ASSIGNMENT((#3829)) ;
#3829=SURFACE_STYLE_USAGE(.BOTH.,#3831) ;
#3831=SURFACE_SIDE_STYLE('',(#3833)) ;
#3833=SURFACE_STYLE_FILL_AREA(#3835) ;
#3835=FILL_AREA_STYLE('Opaque(179,179,179)',(#3837)) ;
#3837=FILL_AREA_STYLE_COLOUR('Opaque(179,179,179)',#3839) ;
#3839=COLOUR_RGB('Opaque(179,179,179)', 0.09019608, 0.27058824, 0.51372549) ;
ENDSEC;
END-ISO-10303-21;
